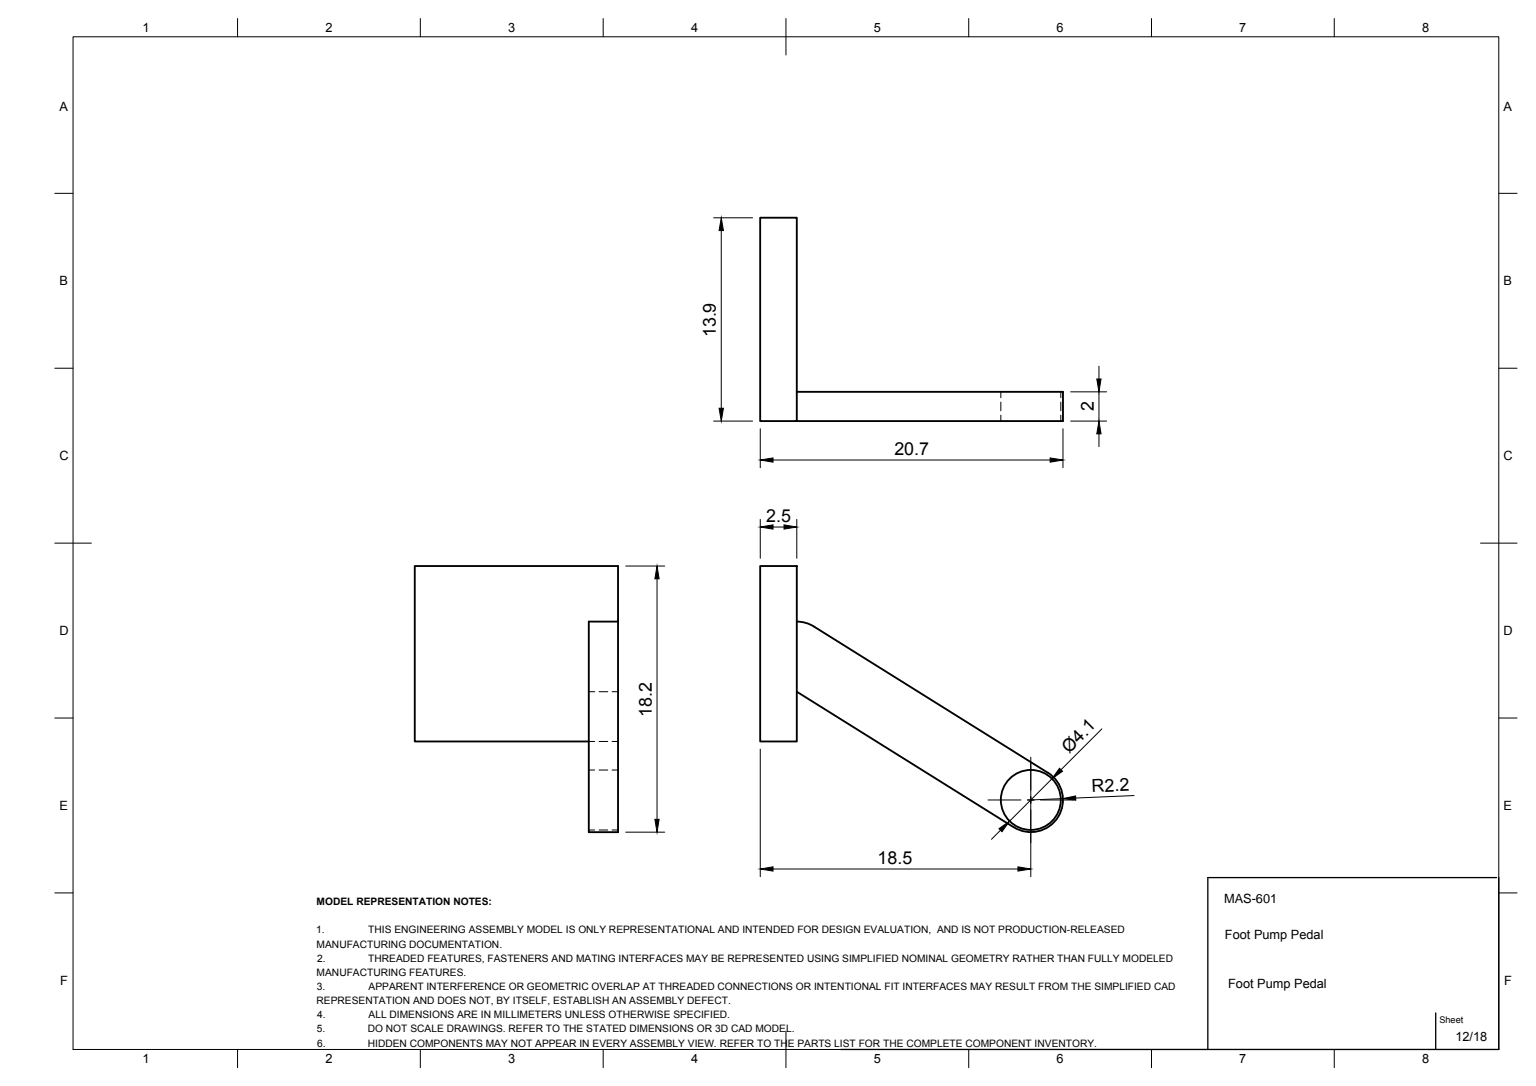
ISO-10303-21;
HEADER;
FILE_DESCRIPTION((''),'2;1');
FILE_NAME('Foot Pump Pedal.step','2026-10-06T07:37:42+05:00',(''),(''),'','','');
FILE_SCHEMA (('AUTOMOTIVE_DESIGN { 1 0 10303 214 3 1 1 }'));
ENDSEC;
DATA;
#10=MECHANICAL_DESIGN_GEOMETRIC_PRESENTATION_REPRESENTATION('',(#380),#18757);
#346=SHAPE_REPRESENTATION_RELATIONSHIP('SRR','None',#18864,#363) ;
#363=ADVANCED_BREP_SHAPE_REPRESENTATION('',(#397),#18747) ;
#380=STYLED_ITEM('',(#18958),#397) ;
#397=MANIFOLD_SOLID_BREP('Foot Pump Pedal',#9549) ;
#576=CYLINDRICAL_SURFACE('',#10163,2.05) ;
#577=CYLINDRICAL_SURFACE('',#10165,2.2) ;
#578=CYLINDRICAL_SURFACE('',#10168,2.19999999999999) ;
#720=FACE_BOUND('',#1903,.T.) ;
#721=FACE_BOUND('',#1910,.T.) ;
#884=PLANE('',#10153) ;
#885=PLANE('',#10154) ;
#886=PLANE('',#10155) ;
#887=PLANE('',#10156) ;
#888=PLANE('',#10157) ;
#889=PLANE('',#10158) ;
#890=PLANE('',#10162) ;
#891=PLANE('',#10167) ;
#892=PLANE('',#10170) ;
#1309=FACE_OUTER_BOUND('',#1897,.T.) ;
#1310=FACE_OUTER_BOUND('',#1898,.T.) ;
#1311=FACE_OUTER_BOUND('',#1899,.T.) ;
#1312=FACE_OUTER_BOUND('',#1900,.T.) ;
#1313=FACE_OUTER_BOUND('',#1901,.T.) ;
#1314=FACE_OUTER_BOUND('',#1902,.T.) ;
#1315=FACE_OUTER_BOUND('',#1904,.T.) ;
#1316=FACE_OUTER_BOUND('',#1905,.T.) ;
#1317=FACE_OUTER_BOUND('',#1906,.T.) ;
#1318=FACE_OUTER_BOUND('',#1907,.T.) ;
#1319=FACE_OUTER_BOUND('',#1908,.T.) ;
#1320=FACE_OUTER_BOUND('',#1909,.T.) ;
#1897=EDGE_LOOP('',(#7451,#7452,#7453,#7454)) ;
#1898=EDGE_LOOP('',(#7455,#7456,#7457,#7458)) ;
#1899=EDGE_LOOP('',(#7459,#7460,#7461,#7462)) ;
#1900=EDGE_LOOP('',(#7463,#7464,#7465,#7466,#7467,#7468,#7469,#7470)) ;
#1901=EDGE_LOOP('',(#7471,#7472,#7473,#7474)) ;
#1902=EDGE_LOOP('',(#7475,#7476,#7477,#7478,#7479)) ;
#1903=EDGE_LOOP('',(#7480)) ;
#1904=EDGE_LOOP('',(#7481,#7482,#7483,#7484)) ;
#1905=EDGE_LOOP('',(#7485,#7486,#7487,#7488)) ;
#1906=EDGE_LOOP('',(#7489,#7490,#7491,#7492)) ;
#1907=EDGE_LOOP('',(#7493,#7494,#7495,#7496)) ;
#1908=EDGE_LOOP('',(#7497,#7498,#7499,#7500)) ;
#1909=EDGE_LOOP('',(#7501,#7502,#7503,#7504,#7505,#7506,#7507,#7508,#7509)) ;
#1910=EDGE_LOOP('',(#7510)) ;
#2589=LINE('',#14863,#3360) ;
#2590=LINE('',#14865,#3361) ;
#2591=LINE('',#14867,#3362) ;
#2592=LINE('',#14868,#3363) ;
#2593=LINE('',#14871,#3364) ;
#2594=LINE('',#14873,#3365) ;
#2595=LINE('',#14874,#3366) ;
#2596=LINE('',#14877,#3367) ;
#2597=LINE('',#14879,#3368) ;
#2598=LINE('',#14880,#3369) ;
#2599=LINE('',#14884,#3370) ;
#2600=LINE('',#14885,#3371) ;
#2601=LINE('',#14887,#3372) ;
#2602=LINE('',#14889,#3373) ;
#2603=LINE('',#14890,#3374) ;
#2604=LINE('',#14892,#3375) ;
#2605=LINE('',#14895,#3376) ;
#2606=LINE('',#14899,#3377) ;
#2607=LINE('',#14905,#3378) ;
#2608=LINE('',#14906,#3379) ;
#2609=LINE('',#14909,#3380) ;
#2610=LINE('',#14913,#3381) ;
#2611=LINE('',#14917,#3382) ;
#2612=LINE('',#14918,#3383) ;
#3360=VECTOR('',#11885,10.) ;
#3361=VECTOR('',#11886,10.) ;
#3362=VECTOR('',#11887,10.) ;
#3363=VECTOR('',#11888,10.) ;
#3364=VECTOR('',#11891,10.) ;
#3365=VECTOR('',#11892,10.) ;
#3366=VECTOR('',#11893,10.) ;
#3367=VECTOR('',#11896,10.) ;
#3368=VECTOR('',#11897,10.) ;
#3369=VECTOR('',#11898,10.) ;
#3370=VECTOR('',#11901,10.) ;
#3371=VECTOR('',#11902,10.) ;
#3372=VECTOR('',#11903,10.) ;
#3373=VECTOR('',#11904,10.) ;
#3374=VECTOR('',#11905,10.) ;
#3375=VECTOR('',#11908,10.) ;
#3376=VECTOR('',#11911,10.) ;
#3377=VECTOR('',#11914,10.) ;
#3378=VECTOR('',#11921,10.) ;
#3379=VECTOR('',#11922,10.) ;
#3380=VECTOR('',#11925,2.05) ;
#3381=VECTOR('',#11930,10.) ;
#3382=VECTOR('',#11935,10.) ;
#3383=VECTOR('',#11936,10.) ;
#3950=CIRCLE('',#10159,2.19999999999999) ;
#3951=CIRCLE('',#10160,2.2) ;
#3952=CIRCLE('',#10161,2.05) ;
#3953=CIRCLE('',#10164,2.05) ;
#3954=CIRCLE('',#10166,2.2) ;
#3955=CIRCLE('',#10169,2.19999999999999) ;
#4513=VERTEX_POINT('',#14861) ;
#4514=VERTEX_POINT('',#14862) ;
#4515=VERTEX_POINT('',#14864) ;
#4516=VERTEX_POINT('',#14866) ;
#4517=VERTEX_POINT('',#14870) ;
#4518=VERTEX_POINT('',#14872) ;
#4519=VERTEX_POINT('',#14876) ;
#4520=VERTEX_POINT('',#14878) ;
#4521=VERTEX_POINT('',#14882) ;
#4522=VERTEX_POINT('',#14883) ;
#4523=VERTEX_POINT('',#14886) ;
#4524=VERTEX_POINT('',#14888) ;
#4525=VERTEX_POINT('',#14894) ;
#4526=VERTEX_POINT('',#14896) ;
#4527=VERTEX_POINT('',#14898) ;
#4528=VERTEX_POINT('',#14901) ;
#4529=VERTEX_POINT('',#14904) ;
#4530=VERTEX_POINT('',#14908) ;
#4531=VERTEX_POINT('',#14912) ;
#4532=VERTEX_POINT('',#14916) ;
#5572=EDGE_CURVE('',#4513,#4514,#2589,.T.) ;
#5573=EDGE_CURVE('',#4514,#4515,#2590,.T.) ;
#5574=EDGE_CURVE('',#4516,#4515,#2591,.T.) ;
#5575=EDGE_CURVE('',#4513,#4516,#2592,.T.) ;
#5576=EDGE_CURVE('',#4517,#4513,#2593,.T.) ;
#5577=EDGE_CURVE('',#4518,#4516,#2594,.T.) ;
#5578=EDGE_CURVE('',#4517,#4518,#2595,.T.) ;
#5579=EDGE_CURVE('',#4514,#4519,#2596,.T.) ;
#5580=EDGE_CURVE('',#4519,#4520,#2597,.T.) ;
#5581=EDGE_CURVE('',#4515,#4520,#2598,.T.) ;
#5582=EDGE_CURVE('',#4521,#4522,#2599,.T.) ;
#5583=EDGE_CURVE('',#4521,#4518,#2600,.T.) ;
#5584=EDGE_CURVE('',#4520,#4523,#2601,.T.) ;
#5585=EDGE_CURVE('',#4524,#4523,#2602,.T.) ;
#5586=EDGE_CURVE('',#4522,#4524,#2603,.T.) ;
#5587=EDGE_CURVE('',#4519,#4517,#2604,.T.) ;
#5588=EDGE_CURVE('',#4524,#4525,#2605,.T.) ;
#5589=EDGE_CURVE('',#4525,#4526,#3950,.T.) ;
#5590=EDGE_CURVE('',#4526,#4527,#2606,.T.) ;
#5591=EDGE_CURVE('',#4527,#4522,#3951,.T.) ;
#5592=EDGE_CURVE('',#4528,#4528,#3952,.T.) ;
#5593=EDGE_CURVE('',#4523,#4529,#2607,.T.) ;
#5594=EDGE_CURVE('',#4529,#4525,#2608,.T.) ;
#5595=EDGE_CURVE('',#4528,#4530,#2609,.T.) ;
#5596=EDGE_CURVE('',#4530,#4530,#3953,.T.) ;
#5597=EDGE_CURVE('',#4531,#4527,#2610,.T.) ;
#5598=EDGE_CURVE('',#4531,#4521,#3954,.T.) ;
#5599=EDGE_CURVE('',#4532,#4531,#2611,.T.) ;
#5600=EDGE_CURVE('',#4532,#4526,#2612,.T.) ;
#5601=EDGE_CURVE('',#4529,#4532,#3955,.T.) ;
#7451=ORIENTED_EDGE('',*,*,#5572,.T.) ;
#7452=ORIENTED_EDGE('',*,*,#5573,.T.) ;
#7453=ORIENTED_EDGE('',*,*,#5574,.F.) ;
#7454=ORIENTED_EDGE('',*,*,#5575,.F.) ;
#7455=ORIENTED_EDGE('',*,*,#5576,.T.) ;
#7456=ORIENTED_EDGE('',*,*,#5575,.T.) ;
#7457=ORIENTED_EDGE('',*,*,#5577,.F.) ;
#7458=ORIENTED_EDGE('',*,*,#5578,.F.) ;
#7459=ORIENTED_EDGE('',*,*,#5579,.T.) ;
#7460=ORIENTED_EDGE('',*,*,#5580,.T.) ;
#7461=ORIENTED_EDGE('',*,*,#5581,.F.) ;
#7462=ORIENTED_EDGE('',*,*,#5573,.F.) ;
#7463=ORIENTED_EDGE('',*,*,#5582,.F.) ;
#7464=ORIENTED_EDGE('',*,*,#5583,.T.) ;
#7465=ORIENTED_EDGE('',*,*,#5577,.T.) ;
#7466=ORIENTED_EDGE('',*,*,#5574,.T.) ;
#7467=ORIENTED_EDGE('',*,*,#5581,.T.) ;
#7468=ORIENTED_EDGE('',*,*,#5584,.T.) ;
#7469=ORIENTED_EDGE('',*,*,#5585,.F.) ;
#7470=ORIENTED_EDGE('',*,*,#5586,.F.) ;
#7471=ORIENTED_EDGE('',*,*,#5579,.F.) ;
#7472=ORIENTED_EDGE('',*,*,#5572,.F.) ;
#7473=ORIENTED_EDGE('',*,*,#5576,.F.) ;
#7474=ORIENTED_EDGE('',*,*,#5587,.F.) ;
#7475=ORIENTED_EDGE('',*,*,#5586,.T.) ;
#7476=ORIENTED_EDGE('',*,*,#5588,.T.) ;
#7477=ORIENTED_EDGE('',*,*,#5589,.T.) ;
#7478=ORIENTED_EDGE('',*,*,#5590,.T.) ;
#7479=ORIENTED_EDGE('',*,*,#5591,.T.) ;
#7480=ORIENTED_EDGE('',*,*,#5592,.T.) ;
#7481=ORIENTED_EDGE('',*,*,#5585,.T.) ;
#7482=ORIENTED_EDGE('',*,*,#5593,.T.) ;
#7483=ORIENTED_EDGE('',*,*,#5594,.T.) ;
#7484=ORIENTED_EDGE('',*,*,#5588,.F.) ;
#7485=ORIENTED_EDGE('',*,*,#5592,.F.) ;
#7486=ORIENTED_EDGE('',*,*,#5595,.T.) ;
#7487=ORIENTED_EDGE('',*,*,#5596,.T.) ;
#7488=ORIENTED_EDGE('',*,*,#5595,.F.) ;
#7489=ORIENTED_EDGE('',*,*,#5582,.T.) ;
#7490=ORIENTED_EDGE('',*,*,#5591,.F.) ;
#7491=ORIENTED_EDGE('',*,*,#5597,.F.) ;
#7492=ORIENTED_EDGE('',*,*,#5598,.T.) ;
#7493=ORIENTED_EDGE('',*,*,#5599,.T.) ;
#7494=ORIENTED_EDGE('',*,*,#5597,.T.) ;
#7495=ORIENTED_EDGE('',*,*,#5590,.F.) ;
#7496=ORIENTED_EDGE('',*,*,#5600,.F.) ;
#7497=ORIENTED_EDGE('',*,*,#5601,.T.) ;
#7498=ORIENTED_EDGE('',*,*,#5600,.T.) ;
#7499=ORIENTED_EDGE('',*,*,#5589,.F.) ;
#7500=ORIENTED_EDGE('',*,*,#5594,.F.) ;
#7501=ORIENTED_EDGE('',*,*,#5598,.F.) ;
#7502=ORIENTED_EDGE('',*,*,#5599,.F.) ;
#7503=ORIENTED_EDGE('',*,*,#5601,.F.) ;
#7504=ORIENTED_EDGE('',*,*,#5593,.F.) ;
#7505=ORIENTED_EDGE('',*,*,#5584,.F.) ;
#7506=ORIENTED_EDGE('',*,*,#5580,.F.) ;
#7507=ORIENTED_EDGE('',*,*,#5587,.T.) ;
#7508=ORIENTED_EDGE('',*,*,#5578,.T.) ;
#7509=ORIENTED_EDGE('',*,*,#5583,.F.) ;
#7510=ORIENTED_EDGE('',*,*,#5596,.F.) ;
#9245=ADVANCED_FACE('',(#1309),#884,.T.) ;
#9246=ADVANCED_FACE('',(#1310),#885,.T.) ;
#9247=ADVANCED_FACE('',(#1311),#886,.T.) ;
#9248=ADVANCED_FACE('',(#1312),#887,.T.) ;
#9249=ADVANCED_FACE('',(#1313),#888,.F.) ;
#9250=ADVANCED_FACE('',(#1314,#720),#889,.T.) ;
#9251=ADVANCED_FACE('',(#1315),#890,.T.) ;
#9252=ADVANCED_FACE('',(#1316),#576,.F.) ;
#9253=ADVANCED_FACE('',(#1317),#577,.T.) ;
#9254=ADVANCED_FACE('',(#1318),#891,.T.) ;
#9255=ADVANCED_FACE('',(#1319),#578,.T.) ;
#9256=ADVANCED_FACE('',(#1320,#721),#892,.F.) ;
#9549=CLOSED_SHELL('',(#9245,#9246,#9247,#9248,#9249,#9250,#9251,#9252,
#9253,#9254,#9255,#9256)) ;
#10152=AXIS2_PLACEMENT_3D('',#14859,#11881,#11882) ;
#10153=AXIS2_PLACEMENT_3D('',#14860,#11883,#11884) ;
#10154=AXIS2_PLACEMENT_3D('',#14869,#11889,#11890) ;
#10155=AXIS2_PLACEMENT_3D('',#14875,#11894,#11895) ;
#10156=AXIS2_PLACEMENT_3D('',#14881,#11899,#11900) ;
#10157=AXIS2_PLACEMENT_3D('',#14891,#11906,#11907) ;
#10158=AXIS2_PLACEMENT_3D('',#14893,#11909,#11910) ;
#10159=AXIS2_PLACEMENT_3D('',#14897,#11912,#11913) ;
#10160=AXIS2_PLACEMENT_3D('',#14900,#11915,#11916) ;
#10161=AXIS2_PLACEMENT_3D('',#14902,#11917,#11918) ;
#10162=AXIS2_PLACEMENT_3D('',#14903,#11919,#11920) ;
#10163=AXIS2_PLACEMENT_3D('',#14907,#11923,#11924) ;
#10164=AXIS2_PLACEMENT_3D('',#14910,#11926,#11927) ;
#10165=AXIS2_PLACEMENT_3D('',#14911,#11928,#11929) ;
#10166=AXIS2_PLACEMENT_3D('',#14914,#11931,#11932) ;
#10167=AXIS2_PLACEMENT_3D('',#14915,#11933,#11934) ;
#10168=AXIS2_PLACEMENT_3D('',#14919,#11937,#11938) ;
#10169=AXIS2_PLACEMENT_3D('',#14920,#11939,#11940) ;
#10170=AXIS2_PLACEMENT_3D('',#14921,#11941,#11942) ;
#11881=DIRECTION('axis',(0.,0.,1.)) ;
#11882=DIRECTION('refdir',(1.,0.,0.)) ;
#11883=DIRECTION('center_axis',(0.,1.,0.)) ;
#11884=DIRECTION('ref_axis',(-1.,0.,0.)) ;
#11885=DIRECTION('',(-1.,0.,0.)) ;
#11886=DIRECTION('',(0.,0.,1.)) ;
#11887=DIRECTION('',(-1.,0.,0.)) ;
#11888=DIRECTION('',(0.,0.,1.)) ;
#11889=DIRECTION('center_axis',(1.,0.,0.)) ;
#11890=DIRECTION('ref_axis',(0.,1.,0.)) ;
#11891=DIRECTION('',(0.,1.,0.)) ;
#11892=DIRECTION('',(0.,1.,0.)) ;
#11893=DIRECTION('',(0.,0.,1.)) ;
#11894=DIRECTION('center_axis',(-1.,0.,0.)) ;
#11895=DIRECTION('ref_axis',(0.,-1.,0.)) ;
#11896=DIRECTION('',(0.,-1.,0.)) ;
#11897=DIRECTION('',(0.,0.,1.)) ;
#11898=DIRECTION('',(0.,-1.,0.)) ;
#11899=DIRECTION('center_axis',(0.,0.,1.)) ;
#11900=DIRECTION('ref_axis',(1.,0.,0.)) ;
#11901=DIRECTION('',(0.,1.,0.)) ;
#11902=DIRECTION('',(1.,0.,0.)) ;
#11903=DIRECTION('',(1.,0.,0.)) ;
#11904=DIRECTION('',(0.,-1.,0.)) ;
#11905=DIRECTION('',(-1.,0.,0.)) ;
#11906=DIRECTION('center_axis',(0.,0.,1.)) ;
#11907=DIRECTION('ref_axis',(1.,0.,0.)) ;
#11908=DIRECTION('',(1.,0.,0.)) ;
#11909=DIRECTION('center_axis',(0.,1.,0.)) ;
#11910=DIRECTION('ref_axis',(1.,0.,0.)) ;
#11911=DIRECTION('',(-0.52999894000318,0.,0.847998304005088)) ;
#11912=DIRECTION('center_axis',(0.,1.,0.)) ;
#11913=DIRECTION('ref_axis',(-0.847998304005088,0.,-0.529998940003181)) ;
#11914=DIRECTION('',(0.52999894000318,0.,-0.847998304005088)) ;
#11915=DIRECTION('center_axis',(0.,1.,0.)) ;
#11916=DIRECTION('ref_axis',(0.847998304005085,0.,0.529998940003185)) ;
#11917=DIRECTION('center_axis',(0.,-1.,0.)) ;
#11918=DIRECTION('ref_axis',(1.,0.,0.)) ;
#11919=DIRECTION('center_axis',(-0.847998304005088,0.,-0.52999894000318)) ;
#11920=DIRECTION('ref_axis',(-0.52999894000318,0.,0.847998304005088)) ;
#11921=DIRECTION('',(-0.52999894000318,0.,0.847998304005088)) ;
#11922=DIRECTION('',(0.,1.,0.)) ;
#11923=DIRECTION('center_axis',(0.,1.,0.)) ;
#11924=DIRECTION('ref_axis',(1.,0.,0.)) ;
#11925=DIRECTION('',(0.,-1.,0.)) ;
#11926=DIRECTION('center_axis',(0.,-1.,0.)) ;
#11927=DIRECTION('ref_axis',(1.,0.,0.)) ;
#11928=DIRECTION('center_axis',(0.,1.,0.)) ;
#11929=DIRECTION('ref_axis',(0.847998304005085,0.,0.529998940003185)) ;
#11930=DIRECTION('',(0.,1.,0.)) ;
#11931=DIRECTION('center_axis',(0.,1.,0.)) ;
#11932=DIRECTION('ref_axis',(0.847998304005085,0.,0.529998940003185)) ;
#11933=DIRECTION('center_axis',(0.847998304005088,0.,0.52999894000318)) ;
#11934=DIRECTION('ref_axis',(0.52999894000318,0.,-0.847998304005088)) ;
#11935=DIRECTION('',(0.52999894000318,0.,-0.847998304005088)) ;
#11936=DIRECTION('',(0.,1.,0.)) ;
#11937=DIRECTION('center_axis',(0.,1.,0.)) ;
#11938=DIRECTION('ref_axis',(-0.847998304005088,0.,-0.529998940003181)) ;
#11939=DIRECTION('center_axis',(0.,1.,0.)) ;
#11940=DIRECTION('ref_axis',(-0.847998304005088,0.,-0.529998940003181)) ;
#11941=DIRECTION('center_axis',(0.,1.,0.)) ;
#11942=DIRECTION('ref_axis',(1.,0.,0.)) ;
#14859=CARTESIAN_POINT('',(0.,0.,0.)) ;
#14860=CARTESIAN_POINT('Origin',(112.,19.,33.5)) ;
#14861=CARTESIAN_POINT('',(112.,19.,33.5)) ;
#14862=CARTESIAN_POINT('',(100.,19.,33.5)) ;
#14863=CARTESIAN_POINT('',(112.,19.,33.5)) ;
#14864=CARTESIAN_POINT('',(100.,19.,36.)) ;
#14865=CARTESIAN_POINT('',(100.,19.,33.5)) ;
#14866=CARTESIAN_POINT('',(112.,19.,36.)) ;
#14867=CARTESIAN_POINT('',(112.,19.,36.)) ;
#14868=CARTESIAN_POINT('',(112.,19.,33.5)) ;
#14869=CARTESIAN_POINT('Origin',(112.,5.1,33.5)) ;
#14870=CARTESIAN_POINT('',(112.,5.1,33.5)) ;
#14871=CARTESIAN_POINT('',(112.,5.1,33.5)) ;
#14872=CARTESIAN_POINT('',(112.,5.1,36.)) ;
#14873=CARTESIAN_POINT('',(112.,5.1,36.)) ;
#14874=CARTESIAN_POINT('',(112.,5.1,33.5)) ;
#14875=CARTESIAN_POINT('Origin',(100.,19.,33.5)) ;
#14876=CARTESIAN_POINT('',(100.,5.1,33.5)) ;
#14877=CARTESIAN_POINT('',(100.,19.,33.5)) ;
#14878=CARTESIAN_POINT('',(100.,5.1,36.)) ;
#14879=CARTESIAN_POINT('',(100.,5.1,33.5)) ;
#14880=CARTESIAN_POINT('',(100.,19.,36.)) ;
#14881=CARTESIAN_POINT('Origin',(106.,12.05,36.)) ;
#14882=CARTESIAN_POINT('',(108.2,5.1,36.)) ;
#14883=CARTESIAN_POINT('',(108.2,7.1,36.)) ;
#14884=CARTESIAN_POINT('',(108.2,5.1,36.)) ;
#14885=CARTESIAN_POINT('',(100.,5.1,36.)) ;
#14886=CARTESIAN_POINT('',(103.405655188684,5.1,36.)) ;
#14887=CARTESIAN_POINT('',(100.,5.1,36.)) ;
#14888=CARTESIAN_POINT('',(103.405655188684,7.1,36.)) ;
#14889=CARTESIAN_POINT('',(103.405655188684,8.575,36.)) ;
#14890=CARTESIAN_POINT('',(103.5,7.1,36.)) ;
#14891=CARTESIAN_POINT('Origin',(106.,12.05,33.5)) ;
#14892=CARTESIAN_POINT('',(100.,5.1,33.5)) ;
#14893=CARTESIAN_POINT('Origin',(101.,7.1,44.)) ;
#14894=CARTESIAN_POINT('',(94.1344037311888,7.1,50.834002331993)) ;
#14895=CARTESIAN_POINT('',(104.134403731189,7.1,34.834002331993)) ;
#14896=CARTESIAN_POINT('',(97.8655962688112,7.1,53.165997668007)) ;
#14897=CARTESIAN_POINT('Origin',(96.,7.1,52.)) ;
#14898=CARTESIAN_POINT('',(107.865596268811,7.1,37.165997668007)) ;
#14899=CARTESIAN_POINT('',(97.8655962688112,7.1,53.165997668007)) ;
#14900=CARTESIAN_POINT('Origin',(106.,7.1,36.)) ;
#14901=CARTESIAN_POINT('',(93.95,7.1,52.)) ;
#14902=CARTESIAN_POINT('Origin',(96.,7.1,52.)) ;
#14903=CARTESIAN_POINT('Origin',(104.134403731189,5.1,34.834002331993)) ;
#14904=CARTESIAN_POINT('',(94.1344037311888,5.1,50.834002331993)) ;
#14905=CARTESIAN_POINT('',(104.134403731189,5.1,34.834002331993)) ;
#14906=CARTESIAN_POINT('',(94.1344037311888,5.1,50.834002331993)) ;
#14907=CARTESIAN_POINT('Origin',(96.,5.1,52.)) ;
#14908=CARTESIAN_POINT('',(93.95,5.1,52.)) ;
#14909=CARTESIAN_POINT('',(93.95,5.1,52.)) ;
#14910=CARTESIAN_POINT('Origin',(96.,5.1,52.)) ;
#14911=CARTESIAN_POINT('Origin',(106.,5.1,36.)) ;
#14912=CARTESIAN_POINT('',(107.865596268811,5.1,37.165997668007)) ;
#14913=CARTESIAN_POINT('',(107.865596268811,5.1,37.165997668007)) ;
#14914=CARTESIAN_POINT('Origin',(106.,5.1,36.)) ;
#14915=CARTESIAN_POINT('Origin',(97.8655962688112,5.1,53.165997668007)) ;
#14916=CARTESIAN_POINT('',(97.8655962688112,5.1,53.165997668007)) ;
#14917=CARTESIAN_POINT('',(97.8655962688112,5.1,53.165997668007)) ;
#14918=CARTESIAN_POINT('',(97.8655962688112,5.1,53.165997668007)) ;
#14919=CARTESIAN_POINT('Origin',(96.,5.1,52.)) ;
#14920=CARTESIAN_POINT('Origin',(96.,5.1,52.)) ;
#14921=CARTESIAN_POINT('Origin',(101.,5.1,44.)) ;
#18728=UNCERTAINTY_MEASURE_WITH_UNIT(LENGTH_MEASURE(0.01),#18758,
'DISTANCE_ACCURACY_VALUE',
'Maximum model space distance between geometric entities at asserted c
onnectivities') ;
#18738=UNCERTAINTY_MEASURE_WITH_UNIT(LENGTH_MEASURE(0.01),#18758,
'DISTANCE_ACCURACY_VALUE',
'Maximum model space distance between geometric entities at asserted c
onnectivities') ;
#18747=(
GEOMETRIC_REPRESENTATION_CONTEXT(3)
GLOBAL_UNCERTAINTY_ASSIGNED_CONTEXT((#18728))
GLOBAL_UNIT_ASSIGNED_CONTEXT((#18758,#18760,#18761))
REPRESENTATION_CONTEXT('','3D')
) ;
#18757=(
GEOMETRIC_REPRESENTATION_CONTEXT(3)
GLOBAL_UNCERTAINTY_ASSIGNED_CONTEXT((#18738))
GLOBAL_UNIT_ASSIGNED_CONTEXT((#18758,#18760,#18761))
REPRESENTATION_CONTEXT('','3D')
) ;
#18758=(
LENGTH_UNIT()
NAMED_UNIT(*)
SI_UNIT(.MILLI.,.METRE.)
) ;
#18760=(
NAMED_UNIT(*)
PLANE_ANGLE_UNIT()
SI_UNIT($,.RADIAN.)
) ;
#18761=(
NAMED_UNIT(*)
SI_UNIT($,.STERADIAN.)
SOLID_ANGLE_UNIT()
) ;
#18770=SHAPE_DEFINITION_REPRESENTATION(#18788,#18864) ;
#18788=PRODUCT_DEFINITION_SHAPE('',$,#18883) ;
#18864=SHAPE_REPRESENTATION('',(#10152),#18747) ;
#18874=PRODUCT_DEFINITION_CONTEXT('part definition',#18930,'design') ;
#18883=PRODUCT_DEFINITION('Foot Pump Pedal','Foot Pump Pedal',#18901,
#18874) ;
#18901=PRODUCT_DEFINITION_FORMATION('',$,#18940) ;
#18930=APPLICATION_CONTEXT(
'Core Data for Automotive Mechanical Design Process') ;
#18931=PRODUCT_CONTEXT('part definition',#18930,'mechanical') ;
#18940=PRODUCT('Foot Pump Pedal','Foot Pump Pedal',$,(#18931)) ;
#18958=PRESENTATION_STYLE_ASSIGNMENT((#18976)) ;
#18976=SURFACE_STYLE_USAGE(.BOTH.,#18994) ;
#18994=SURFACE_SIDE_STYLE('',(#19012)) ;
#19012=SURFACE_STYLE_FILL_AREA(#19030) ;
#19030=FILL_AREA_STYLE('MAS-253 Metallic Sheet - Foot Pump Pedal',(#19048)) ;
#19048=FILL_AREA_STYLE_COLOUR(
'MAS-253 Metallic Sheet - Foot Pump Pedal',#19066) ;
#19066=COLOUR_RGB('MAS-253 Metallic Sheet - Foot Pump Pedal', 0.31764706, 0.68627451, 0.89019608) ;
ENDSEC;
END-ISO-10303-21;
